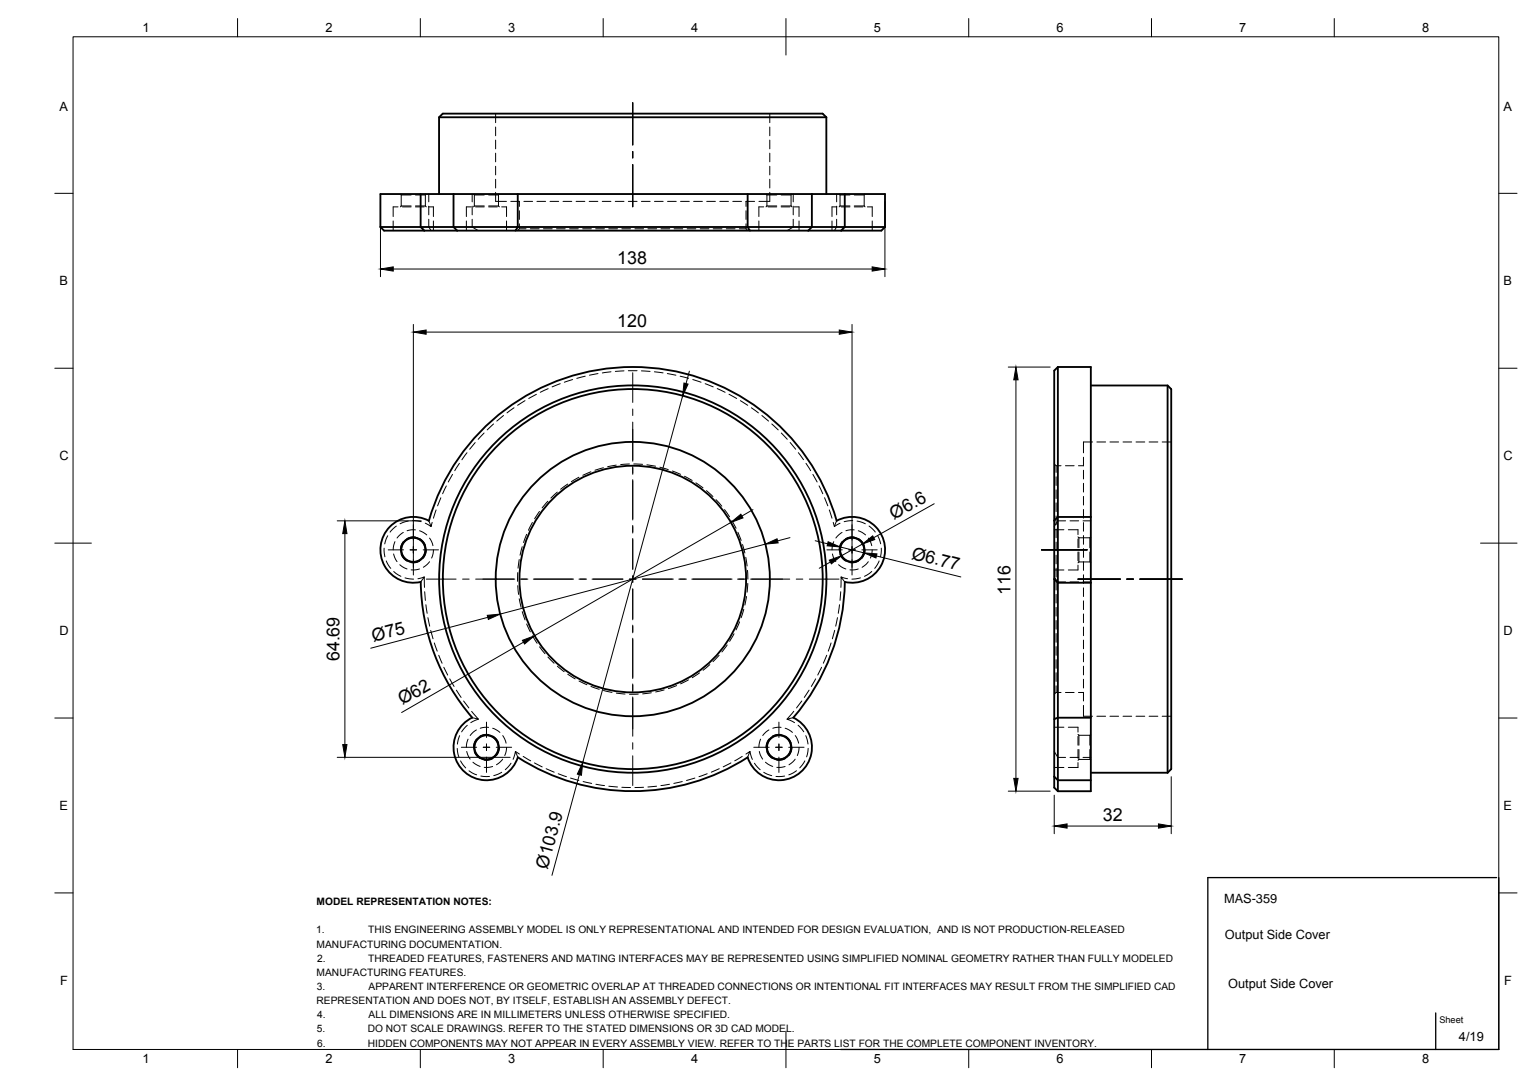
ISO-10303-21;
HEADER;
/* Generated by software containing ST-Developer
 * from STEP Tools, Inc. (www.steptools.com) 
 */

FILE_DESCRIPTION(
/* description */ (''),
/* implementation_level */ '2;1');

FILE_NAME(
/* name */ 'Output Side Cover.step',
/* time_stamp */ '2026-10-15T14:25:16-07:00',
/* author */ (''),
/* organization */ (''),
/* preprocessor_version */ 'ST-DEVELOPER v20.2',
/* originating_system */ 'Autodesk Translation Framework v15.15.0.0',
/* authorisation */ '');

FILE_SCHEMA (('AUTOMOTIVE_DESIGN { 1 0 10303 214 3 1 1 }'));
ENDSEC;

DATA;
#10=MECHANICAL_DESIGN_GEOMETRIC_PRESENTATION_REPRESENTATION('',(#324),#86429);
#288=SHAPE_REPRESENTATION_RELATIONSHIP('SRR','None',#86503,#306);
#306=ADVANCED_BREP_SHAPE_REPRESENTATION('',(#342),#86412);
#324=STYLED_ITEM('',(#86602),#342);
#342=MANIFOLD_SOLID_BREP('Body1',#15614);
#387=B_SPLINE_CURVE_WITH_KNOTS('',3,(#22589,#22590,#22591,#22592),
 .UNSPECIFIED.,.F.,.F.,(4,4),(-0.195594022319082,0.),.UNSPECIFIED.);
#388=B_SPLINE_CURVE_WITH_KNOTS('',3,(#22595,#22596,#22597,#22598),
 .UNSPECIFIED.,.F.,.F.,(4,4),(-0.195594022319045,0.),.UNSPECIFIED.);
#389=B_SPLINE_CURVE_WITH_KNOTS('',3,(#22603,#22604,#22605,#22606),
 .UNSPECIFIED.,.F.,.F.,(4,4),(-0.195594022319034,0.),.UNSPECIFIED.);
#390=B_SPLINE_CURVE_WITH_KNOTS('',3,(#22612,#22613,#22614,#22615),
 .UNSPECIFIED.,.F.,.F.,(4,4),(-0.201492965018152,0.),.UNSPECIFIED.);
#391=B_SPLINE_CURVE_WITH_KNOTS('',3,(#22621,#22622,#22623,#22624),
 .UNSPECIFIED.,.F.,.F.,(4,4),(-0.201492965018184,0.),.UNSPECIFIED.);
#392=B_SPLINE_CURVE_WITH_KNOTS('',3,(#22630,#22631,#22632,#22633),
 .UNSPECIFIED.,.F.,.F.,(4,4),(-0.201492965018239,0.),.UNSPECIFIED.);
#393=B_SPLINE_CURVE_WITH_KNOTS('',3,(#22640,#22641,#22642,#22643),
 .UNSPECIFIED.,.F.,.F.,(4,4),(-0.201492965018198,0.),.UNSPECIFIED.);
#394=B_SPLINE_CURVE_WITH_KNOTS('',3,(#22649,#22650,#22651,#22652),
 .UNSPECIFIED.,.F.,.F.,(4,4),(-0.195594022319061,0.),.UNSPECIFIED.);
#1193=CONICAL_SURFACE('',#16204,5.245,0.785398163397446);
#1194=CONICAL_SURFACE('',#16211,5.75,0.785398163397448);
#1195=CONICAL_SURFACE('',#16214,0.85,0.785398163397452);
#1196=CONICAL_SURFACE('',#16217,5.75,0.785398163397448);
#1197=CONICAL_SURFACE('',#16220,0.85,0.785398163397451);
#1198=CONICAL_SURFACE('',#16223,5.75,0.785398163397453);
#1199=CONICAL_SURFACE('',#16226,0.85,0.785398163397449);
#1200=CONICAL_SURFACE('',#16229,5.75,0.785398163397448);
#1201=CONICAL_SURFACE('',#16232,0.85,0.785398163397452);
#1202=CONICAL_SURFACE('',#16249,0.342499999999999,0.32175055439664);
#1203=CONICAL_SURFACE('',#16254,0.342499999999999,0.785398163397439);
#1204=CONICAL_SURFACE('',#16259,0.342499999999999,0.321750554396635);
#1205=CONICAL_SURFACE('',#16264,0.342499999999999,0.785398163397431);
#1206=CONICAL_SURFACE('',#16269,0.342499999999999,0.321750554396635);
#1207=CONICAL_SURFACE('',#16274,0.342499999999999,0.785398163397431);
#1208=CONICAL_SURFACE('',#16279,0.342499999999999,0.321750554396635);
#1209=CONICAL_SURFACE('',#16284,0.342499999999999,0.785398163397431);
#1210=CONICAL_SURFACE('',#16289,3.155,0.785398163397444);
#1399=CYLINDRICAL_SURFACE('',#16207,5.295);
#1400=CYLINDRICAL_SURFACE('',#16235,0.9);
#1401=CYLINDRICAL_SURFACE('',#16237,5.8);
#1402=CYLINDRICAL_SURFACE('',#16239,0.9);
#1403=CYLINDRICAL_SURFACE('',#16241,5.8);
#1404=CYLINDRICAL_SURFACE('',#16252,0.33);
#1405=CYLINDRICAL_SURFACE('',#16258,0.55);
#1406=CYLINDRICAL_SURFACE('',#16262,0.33);
#1407=CYLINDRICAL_SURFACE('',#16268,0.55);
#1408=CYLINDRICAL_SURFACE('',#16272,0.33);
#1409=CYLINDRICAL_SURFACE('',#16278,0.55);
#1410=CYLINDRICAL_SURFACE('',#16282,0.33);
#1411=CYLINDRICAL_SURFACE('',#16288,0.55);
#1412=CYLINDRICAL_SURFACE('',#16291,3.1);
#1413=CYLINDRICAL_SURFACE('',#16295,3.75);
#1414=CYLINDRICAL_SURFACE('',#16296,0.9);
#1415=CYLINDRICAL_SURFACE('',#16298,5.8);
#1416=CYLINDRICAL_SURFACE('',#16300,0.9);
#1417=CYLINDRICAL_SURFACE('',#16302,5.8);
#1652=FACE_BOUND('',#3542,.T.);
#1653=FACE_BOUND('',#3556,.T.);
#1654=FACE_BOUND('',#3557,.T.);
#1655=FACE_BOUND('',#3558,.T.);
#1656=FACE_BOUND('',#3559,.T.);
#1657=FACE_BOUND('',#3560,.T.);
#1658=FACE_BOUND('',#3565,.T.);
#1659=FACE_BOUND('',#3571,.T.);
#1660=FACE_BOUND('',#3577,.T.);
#1661=FACE_BOUND('',#3583,.T.);
#1662=FACE_BOUND('',#3588,.T.);
#1663=FACE_BOUND('',#3595,.T.);
#1664=FACE_BOUND('',#3596,.T.);
#1665=FACE_BOUND('',#3597,.T.);
#1666=FACE_BOUND('',#3598,.T.);
#1667=FACE_BOUND('',#3599,.T.);
#1889=CIRCLE('',#16205,5.295);
#1890=CIRCLE('',#16206,5.195);
#1891=CIRCLE('',#16208,5.295);
#1892=CIRCLE('',#16210,3.75);
#1893=CIRCLE('',#16212,5.7);
#1894=CIRCLE('',#16213,5.8);
#1895=CIRCLE('',#16215,0.8);
#1896=CIRCLE('',#16216,0.9);
#1897=CIRCLE('',#16218,5.7);
#1898=CIRCLE('',#16219,5.8);
#1899=CIRCLE('',#16221,0.8);
#1900=CIRCLE('',#16222,0.9);
#1901=CIRCLE('',#16224,5.7);
#1902=CIRCLE('',#16225,5.8);
#1903=CIRCLE('',#16227,0.9);
#1904=CIRCLE('',#16228,0.8);
#1905=CIRCLE('',#16230,5.8);
#1906=CIRCLE('',#16231,5.7);
#1907=CIRCLE('',#16233,0.9);
#1908=CIRCLE('',#16234,0.8);
#1909=CIRCLE('',#16236,0.9);
#1910=CIRCLE('',#16238,5.8);
#1911=CIRCLE('',#16240,0.9);
#1912=CIRCLE('',#16242,5.8);
#1913=CIRCLE('',#16244,3.15);
#1914=CIRCLE('',#16245,0.55);
#1915=CIRCLE('',#16246,0.55);
#1916=CIRCLE('',#16247,0.55);
#1917=CIRCLE('',#16248,0.55);
#1918=CIRCLE('',#16250,0.33);
#1919=CIRCLE('',#16251,0.338333333333333);
#1920=CIRCLE('',#16253,0.33);
#1921=CIRCLE('',#16255,0.355);
#1922=CIRCLE('',#16257,0.55);
#1923=CIRCLE('',#16260,0.33);
#1924=CIRCLE('',#16261,0.338333333333333);
#1925=CIRCLE('',#16263,0.33);
#1926=CIRCLE('',#16265,0.355);
#1927=CIRCLE('',#16267,0.55);
#1928=CIRCLE('',#16270,0.33);
#1929=CIRCLE('',#16271,0.338333333333333);
#1930=CIRCLE('',#16273,0.33);
#1931=CIRCLE('',#16275,0.355);
#1932=CIRCLE('',#16277,0.55);
#1933=CIRCLE('',#16280,0.33);
#1934=CIRCLE('',#16281,0.338333333333333);
#1935=CIRCLE('',#16283,0.33);
#1936=CIRCLE('',#16285,0.355);
#1937=CIRCLE('',#16287,0.55);
#1938=CIRCLE('',#16290,3.1);
#1939=CIRCLE('',#16292,3.1);
#1940=CIRCLE('',#16294,3.75);
#1941=CIRCLE('',#16297,0.9);
#1942=CIRCLE('',#16299,5.8);
#1943=CIRCLE('',#16301,0.9);
#1944=CIRCLE('',#16303,5.8);
#2617=FACE_OUTER_BOUND('',#3539,.T.);
#2618=FACE_OUTER_BOUND('',#3540,.T.);
#2619=FACE_OUTER_BOUND('',#3541,.T.);
#2620=FACE_OUTER_BOUND('',#3543,.T.);
#2621=FACE_OUTER_BOUND('',#3544,.T.);
#2622=FACE_OUTER_BOUND('',#3545,.T.);
#2623=FACE_OUTER_BOUND('',#3546,.T.);
#2624=FACE_OUTER_BOUND('',#3547,.T.);
#2625=FACE_OUTER_BOUND('',#3548,.T.);
#2626=FACE_OUTER_BOUND('',#3549,.T.);
#2627=FACE_OUTER_BOUND('',#3550,.T.);
#2628=FACE_OUTER_BOUND('',#3551,.T.);
#2629=FACE_OUTER_BOUND('',#3552,.T.);
#2630=FACE_OUTER_BOUND('',#3553,.T.);
#2631=FACE_OUTER_BOUND('',#3554,.T.);
#2632=FACE_OUTER_BOUND('',#3555,.T.);
#2633=FACE_OUTER_BOUND('',#3561,.T.);
#2634=FACE_OUTER_BOUND('',#3562,.T.);
#2635=FACE_OUTER_BOUND('',#3563,.T.);
#2636=FACE_OUTER_BOUND('',#3564,.T.);
#2637=FACE_OUTER_BOUND('',#3566,.T.);
#2638=FACE_OUTER_BOUND('',#3567,.T.);
#2639=FACE_OUTER_BOUND('',#3568,.T.);
#2640=FACE_OUTER_BOUND('',#3569,.T.);
#2641=FACE_OUTER_BOUND('',#3570,.T.);
#2642=FACE_OUTER_BOUND('',#3572,.T.);
#2643=FACE_OUTER_BOUND('',#3573,.T.);
#2644=FACE_OUTER_BOUND('',#3574,.T.);
#2645=FACE_OUTER_BOUND('',#3575,.T.);
#2646=FACE_OUTER_BOUND('',#3576,.T.);
#2647=FACE_OUTER_BOUND('',#3578,.T.);
#2648=FACE_OUTER_BOUND('',#3579,.T.);
#2649=FACE_OUTER_BOUND('',#3580,.T.);
#2650=FACE_OUTER_BOUND('',#3581,.T.);
#2651=FACE_OUTER_BOUND('',#3582,.T.);
#2652=FACE_OUTER_BOUND('',#3584,.T.);
#2653=FACE_OUTER_BOUND('',#3585,.T.);
#2654=FACE_OUTER_BOUND('',#3586,.T.);
#2655=FACE_OUTER_BOUND('',#3587,.T.);
#2656=FACE_OUTER_BOUND('',#3589,.T.);
#2657=FACE_OUTER_BOUND('',#3590,.T.);
#2658=FACE_OUTER_BOUND('',#3591,.T.);
#2659=FACE_OUTER_BOUND('',#3592,.T.);
#2660=FACE_OUTER_BOUND('',#3593,.T.);
#2661=FACE_OUTER_BOUND('',#3594,.T.);
#3539=EDGE_LOOP('',(#11021,#11022,#11023,#11024));
#3540=EDGE_LOOP('',(#11025,#11026,#11027,#11028));
#3541=EDGE_LOOP('',(#11029));
#3542=EDGE_LOOP('',(#11030));
#3543=EDGE_LOOP('',(#11031,#11032,#11033,#11034));
#3544=EDGE_LOOP('',(#11035,#11036,#11037,#11038));
#3545=EDGE_LOOP('',(#11039,#11040,#11041,#11042));
#3546=EDGE_LOOP('',(#11043,#11044,#11045,#11046));
#3547=EDGE_LOOP('',(#11047,#11048,#11049,#11050));
#3548=EDGE_LOOP('',(#11051,#11052,#11053,#11054));
#3549=EDGE_LOOP('',(#11055,#11056,#11057,#11058));
#3550=EDGE_LOOP('',(#11059,#11060,#11061,#11062));
#3551=EDGE_LOOP('',(#11063,#11064,#11065,#11066));
#3552=EDGE_LOOP('',(#11067,#11068,#11069,#11070));
#3553=EDGE_LOOP('',(#11071,#11072,#11073,#11074));
#3554=EDGE_LOOP('',(#11075,#11076,#11077,#11078));
#3555=EDGE_LOOP('',(#11079,#11080,#11081,#11082,#11083,#11084,#11085,#11086));
#3556=EDGE_LOOP('',(#11087));
#3557=EDGE_LOOP('',(#11088));
#3558=EDGE_LOOP('',(#11089));
#3559=EDGE_LOOP('',(#11090));
#3560=EDGE_LOOP('',(#11091));
#3561=EDGE_LOOP('',(#11092,#11093,#11094,#11095));
#3562=EDGE_LOOP('',(#11096,#11097,#11098,#11099));
#3563=EDGE_LOOP('',(#11100,#11101,#11102,#11103));
#3564=EDGE_LOOP('',(#11104));
#3565=EDGE_LOOP('',(#11105));
#3566=EDGE_LOOP('',(#11106,#11107,#11108,#11109));
#3567=EDGE_LOOP('',(#11110,#11111,#11112,#11113));
#3568=EDGE_LOOP('',(#11114,#11115,#11116,#11117));
#3569=EDGE_LOOP('',(#11118,#11119,#11120,#11121));
#3570=EDGE_LOOP('',(#11122));
#3571=EDGE_LOOP('',(#11123));
#3572=EDGE_LOOP('',(#11124,#11125,#11126,#11127));
#3573=EDGE_LOOP('',(#11128,#11129,#11130,#11131));
#3574=EDGE_LOOP('',(#11132,#11133,#11134,#11135));
#3575=EDGE_LOOP('',(#11136,#11137,#11138,#11139));
#3576=EDGE_LOOP('',(#11140));
#3577=EDGE_LOOP('',(#11141));
#3578=EDGE_LOOP('',(#11142,#11143,#11144,#11145));
#3579=EDGE_LOOP('',(#11146,#11147,#11148,#11149));
#3580=EDGE_LOOP('',(#11150,#11151,#11152,#11153));
#3581=EDGE_LOOP('',(#11154,#11155,#11156,#11157));
#3582=EDGE_LOOP('',(#11158));
#3583=EDGE_LOOP('',(#11159));
#3584=EDGE_LOOP('',(#11160,#11161,#11162,#11163));
#3585=EDGE_LOOP('',(#11164,#11165,#11166,#11167));
#3586=EDGE_LOOP('',(#11168,#11169,#11170,#11171));
#3587=EDGE_LOOP('',(#11172));
#3588=EDGE_LOOP('',(#11173));
#3589=EDGE_LOOP('',(#11174,#11175,#11176,#11177));
#3590=EDGE_LOOP('',(#11178,#11179,#11180,#11181));
#3591=EDGE_LOOP('',(#11182,#11183,#11184,#11185));
#3592=EDGE_LOOP('',(#11186,#11187,#11188,#11189));
#3593=EDGE_LOOP('',(#11190,#11191,#11192,#11193));
#3594=EDGE_LOOP('',(#11194,#11195,#11196,#11197,#11198,#11199,#11200,#11201));
#3595=EDGE_LOOP('',(#11202));
#3596=EDGE_LOOP('',(#11203));
#3597=EDGE_LOOP('',(#11204));
#3598=EDGE_LOOP('',(#11205));
#3599=EDGE_LOOP('',(#11206));
#4703=LINE('',#22575,#5563);
#4704=LINE('',#22579,#5564);
#4705=LINE('',#22658,#5565);
#4706=LINE('',#22661,#5566);
#4707=LINE('',#22664,#5567);
#4708=LINE('',#22668,#5568);
#4709=LINE('',#22672,#5569);
#4710=LINE('',#22689,#5570);
#4711=LINE('',#22693,#5571);
#4712=LINE('',#22697,#5572);
#4713=LINE('',#22703,#5573);
#4714=LINE('',#22708,#5574);
#4715=LINE('',#22712,#5575);
#4716=LINE('',#22716,#5576);
#4717=LINE('',#22722,#5577);
#4718=LINE('',#22727,#5578);
#4719=LINE('',#22731,#5579);
#4720=LINE('',#22735,#5580);
#4721=LINE('',#22741,#5581);
#4722=LINE('',#22746,#5582);
#4723=LINE('',#22750,#5583);
#4724=LINE('',#22754,#5584);
#4725=LINE('',#22760,#5585);
#4726=LINE('',#22764,#5586);
#4727=LINE('',#22767,#5587);
#4728=LINE('',#22773,#5588);
#4729=LINE('',#22776,#5589);
#4730=LINE('',#22780,#5590);
#4731=LINE('',#22784,#5591);
#5563=VECTOR('',#18460,5.245);
#5564=VECTOR('',#18465,5.295);
#5565=VECTOR('',#18522,1.);
#5566=VECTOR('',#18525,1.);
#5567=VECTOR('',#18528,1.);
#5568=VECTOR('',#18533,1.);
#5569=VECTOR('',#18538,1.);
#5570=VECTOR('',#18557,0.342499999999999);
#5571=VECTOR('',#18562,0.33);
#5572=VECTOR('',#18567,0.342499999999999);
#5573=VECTOR('',#18576,0.55);
#5574=VECTOR('',#18581,0.342499999999999);
#5575=VECTOR('',#18586,0.33);
#5576=VECTOR('',#18591,0.342499999999999);
#5577=VECTOR('',#18600,0.55);
#5578=VECTOR('',#18605,0.342499999999999);
#5579=VECTOR('',#18610,0.33);
#5580=VECTOR('',#18615,0.342499999999999);
#5581=VECTOR('',#18624,0.55);
#5582=VECTOR('',#18629,0.342499999999999);
#5583=VECTOR('',#18634,0.33);
#5584=VECTOR('',#18639,0.342499999999999);
#5585=VECTOR('',#18648,0.55);
#5586=VECTOR('',#18653,3.155);
#5587=VECTOR('',#18656,3.1);
#5588=VECTOR('',#18665,3.75);
#5589=VECTOR('',#18668,1.);
#5590=VECTOR('',#18673,1.);
#5591=VECTOR('',#18678,1.);
#6386=VERTEX_POINT('',#22572);
#6387=VERTEX_POINT('',#22574);
#6388=VERTEX_POINT('',#22578);
#6389=VERTEX_POINT('',#22582);
#6390=VERTEX_POINT('',#22585);
#6391=VERTEX_POINT('',#22586);
#6392=VERTEX_POINT('',#22588);
#6393=VERTEX_POINT('',#22593);
#6394=VERTEX_POINT('',#22600);
#6395=VERTEX_POINT('',#22602);
#6396=VERTEX_POINT('',#22609);
#6397=VERTEX_POINT('',#22611);
#6398=VERTEX_POINT('',#22618);
#6399=VERTEX_POINT('',#22620);
#6400=VERTEX_POINT('',#22627);
#6401=VERTEX_POINT('',#22629);
#6402=VERTEX_POINT('',#22636);
#6403=VERTEX_POINT('',#22638);
#6404=VERTEX_POINT('',#22645);
#6405=VERTEX_POINT('',#22647);
#6406=VERTEX_POINT('',#22657);
#6407=VERTEX_POINT('',#22659);
#6408=VERTEX_POINT('',#22663);
#6409=VERTEX_POINT('',#22667);
#6410=VERTEX_POINT('',#22671);
#6411=VERTEX_POINT('',#22675);
#6412=VERTEX_POINT('',#22677);
#6413=VERTEX_POINT('',#22679);
#6414=VERTEX_POINT('',#22681);
#6415=VERTEX_POINT('',#22683);
#6416=VERTEX_POINT('',#22686);
#6417=VERTEX_POINT('',#22688);
#6418=VERTEX_POINT('',#22692);
#6419=VERTEX_POINT('',#22696);
#6420=VERTEX_POINT('',#22700);
#6421=VERTEX_POINT('',#22705);
#6422=VERTEX_POINT('',#22707);
#6423=VERTEX_POINT('',#22711);
#6424=VERTEX_POINT('',#22715);
#6425=VERTEX_POINT('',#22719);
#6426=VERTEX_POINT('',#22724);
#6427=VERTEX_POINT('',#22726);
#6428=VERTEX_POINT('',#22730);
#6429=VERTEX_POINT('',#22734);
#6430=VERTEX_POINT('',#22738);
#6431=VERTEX_POINT('',#22743);
#6432=VERTEX_POINT('',#22745);
#6433=VERTEX_POINT('',#22749);
#6434=VERTEX_POINT('',#22753);
#6435=VERTEX_POINT('',#22757);
#6436=VERTEX_POINT('',#22762);
#6437=VERTEX_POINT('',#22766);
#6438=VERTEX_POINT('',#22770);
#6439=VERTEX_POINT('',#22775);
#6440=VERTEX_POINT('',#22779);
#6441=VERTEX_POINT('',#22783);
#8132=EDGE_CURVE('',#6386,#6386,#1889,.T.);
#8133=EDGE_CURVE('',#6386,#6387,#4703,.T.);
#8134=EDGE_CURVE('',#6387,#6387,#1890,.T.);
#8135=EDGE_CURVE('',#6386,#6388,#4704,.T.);
#8136=EDGE_CURVE('',#6388,#6388,#1891,.T.);
#8137=EDGE_CURVE('',#6389,#6389,#1892,.T.);
#8138=EDGE_CURVE('',#6390,#6391,#1893,.T.);
#8139=EDGE_CURVE('',#6391,#6392,#387,.T.);
#8140=EDGE_CURVE('',#6392,#6393,#1894,.T.);
#8141=EDGE_CURVE('',#6390,#6393,#388,.T.);
#8142=EDGE_CURVE('',#6391,#6394,#1895,.T.);
#8143=EDGE_CURVE('',#6394,#6395,#389,.T.);
#8144=EDGE_CURVE('',#6395,#6392,#1896,.T.);
#8145=EDGE_CURVE('',#6394,#6396,#1897,.T.);
#8146=EDGE_CURVE('',#6396,#6397,#390,.T.);
#8147=EDGE_CURVE('',#6397,#6395,#1898,.T.);
#8148=EDGE_CURVE('',#6396,#6398,#1899,.T.);
#8149=EDGE_CURVE('',#6398,#6399,#391,.T.);
#8150=EDGE_CURVE('',#6399,#6397,#1900,.T.);
#8151=EDGE_CURVE('',#6398,#6400,#1901,.T.);
#8152=EDGE_CURVE('',#6400,#6401,#392,.T.);
#8153=EDGE_CURVE('',#6401,#6399,#1902,.T.);
#8154=EDGE_CURVE('',#6402,#6401,#1903,.T.);
#8155=EDGE_CURVE('',#6400,#6403,#1904,.T.);
#8156=EDGE_CURVE('',#6403,#6402,#393,.T.);
#8157=EDGE_CURVE('',#6404,#6402,#1905,.T.);
#8158=EDGE_CURVE('',#6403,#6405,#1906,.T.);
#8159=EDGE_CURVE('',#6405,#6404,#394,.T.);
#8160=EDGE_CURVE('',#6393,#6404,#1907,.T.);
#8161=EDGE_CURVE('',#6405,#6390,#1908,.T.);
#8162=EDGE_CURVE('',#6406,#6402,#4705,.T.);
#8163=EDGE_CURVE('',#6407,#6406,#1909,.T.);
#8164=EDGE_CURVE('',#6407,#6401,#4706,.T.);
#8165=EDGE_CURVE('',#6408,#6404,#4707,.T.);
#8166=EDGE_CURVE('',#6406,#6408,#1910,.T.);
#8167=EDGE_CURVE('',#6409,#6393,#4708,.T.);
#8168=EDGE_CURVE('',#6408,#6409,#1911,.T.);
#8169=EDGE_CURVE('',#6410,#6392,#4709,.T.);
#8170=EDGE_CURVE('',#6409,#6410,#1912,.T.);
#8171=EDGE_CURVE('',#6411,#6411,#1913,.T.);
#8172=EDGE_CURVE('',#6412,#6412,#1914,.T.);
#8173=EDGE_CURVE('',#6413,#6413,#1915,.T.);
#8174=EDGE_CURVE('',#6414,#6414,#1916,.T.);
#8175=EDGE_CURVE('',#6415,#6415,#1917,.T.);
#8176=EDGE_CURVE('',#6416,#6416,#1918,.T.);
#8177=EDGE_CURVE('',#6416,#6417,#4710,.T.);
#8178=EDGE_CURVE('',#6417,#6417,#1919,.T.);
#8179=EDGE_CURVE('',#6416,#6418,#4711,.T.);
#8180=EDGE_CURVE('',#6418,#6418,#1920,.T.);
#8181=EDGE_CURVE('',#6418,#6419,#4712,.T.);
#8182=EDGE_CURVE('',#6419,#6419,#1921,.T.);
#8183=EDGE_CURVE('',#6420,#6420,#1922,.T.);
#8184=EDGE_CURVE('',#6420,#6415,#4713,.T.);
#8185=EDGE_CURVE('',#6421,#6421,#1923,.T.);
#8186=EDGE_CURVE('',#6421,#6422,#4714,.T.);
#8187=EDGE_CURVE('',#6422,#6422,#1924,.T.);
#8188=EDGE_CURVE('',#6421,#6423,#4715,.T.);
#8189=EDGE_CURVE('',#6423,#6423,#1925,.T.);
#8190=EDGE_CURVE('',#6423,#6424,#4716,.T.);
#8191=EDGE_CURVE('',#6424,#6424,#1926,.T.);
#8192=EDGE_CURVE('',#6425,#6425,#1927,.T.);
#8193=EDGE_CURVE('',#6425,#6414,#4717,.T.);
#8194=EDGE_CURVE('',#6426,#6426,#1928,.T.);
#8195=EDGE_CURVE('',#6426,#6427,#4718,.T.);
#8196=EDGE_CURVE('',#6427,#6427,#1929,.T.);
#8197=EDGE_CURVE('',#6426,#6428,#4719,.T.);
#8198=EDGE_CURVE('',#6428,#6428,#1930,.T.);
#8199=EDGE_CURVE('',#6428,#6429,#4720,.T.);
#8200=EDGE_CURVE('',#6429,#6429,#1931,.T.);
#8201=EDGE_CURVE('',#6430,#6430,#1932,.T.);
#8202=EDGE_CURVE('',#6430,#6413,#4721,.T.);
#8203=EDGE_CURVE('',#6431,#6431,#1933,.T.);
#8204=EDGE_CURVE('',#6431,#6432,#4722,.T.);
#8205=EDGE_CURVE('',#6432,#6432,#1934,.T.);
#8206=EDGE_CURVE('',#6431,#6433,#4723,.T.);
#8207=EDGE_CURVE('',#6433,#6433,#1935,.T.);
#8208=EDGE_CURVE('',#6433,#6434,#4724,.T.);
#8209=EDGE_CURVE('',#6434,#6434,#1936,.T.);
#8210=EDGE_CURVE('',#6435,#6435,#1937,.T.);
#8211=EDGE_CURVE('',#6435,#6412,#4725,.T.);
#8212=EDGE_CURVE('',#6436,#6436,#1938,.T.);
#8213=EDGE_CURVE('',#6436,#6411,#4726,.T.);
#8214=EDGE_CURVE('',#6436,#6437,#4727,.T.);
#8215=EDGE_CURVE('',#6437,#6437,#1939,.T.);
#8216=EDGE_CURVE('',#6438,#6438,#1940,.T.);
#8217=EDGE_CURVE('',#6438,#6389,#4728,.T.);
#8218=EDGE_CURVE('',#6439,#6395,#4729,.T.);
#8219=EDGE_CURVE('',#6410,#6439,#1941,.T.);
#8220=EDGE_CURVE('',#6440,#6397,#4730,.T.);
#8221=EDGE_CURVE('',#6439,#6440,#1942,.T.);
#8222=EDGE_CURVE('',#6441,#6399,#4731,.T.);
#8223=EDGE_CURVE('',#6440,#6441,#1943,.T.);
#8224=EDGE_CURVE('',#6441,#6407,#1944,.T.);
#11021=ORIENTED_EDGE('',*,*,#8132,.T.);
#11022=ORIENTED_EDGE('',*,*,#8133,.T.);
#11023=ORIENTED_EDGE('',*,*,#8134,.T.);
#11024=ORIENTED_EDGE('',*,*,#8133,.F.);
#11025=ORIENTED_EDGE('',*,*,#8132,.F.);
#11026=ORIENTED_EDGE('',*,*,#8135,.T.);
#11027=ORIENTED_EDGE('',*,*,#8136,.F.);
#11028=ORIENTED_EDGE('',*,*,#8135,.F.);
#11029=ORIENTED_EDGE('',*,*,#8134,.F.);
#11030=ORIENTED_EDGE('',*,*,#8137,.T.);
#11031=ORIENTED_EDGE('',*,*,#8138,.T.);
#11032=ORIENTED_EDGE('',*,*,#8139,.T.);
#11033=ORIENTED_EDGE('',*,*,#8140,.T.);
#11034=ORIENTED_EDGE('',*,*,#8141,.F.);
#11035=ORIENTED_EDGE('',*,*,#8142,.T.);
#11036=ORIENTED_EDGE('',*,*,#8143,.T.);
#11037=ORIENTED_EDGE('',*,*,#8144,.T.);
#11038=ORIENTED_EDGE('',*,*,#8139,.F.);
#11039=ORIENTED_EDGE('',*,*,#8145,.T.);
#11040=ORIENTED_EDGE('',*,*,#8146,.T.);
#11041=ORIENTED_EDGE('',*,*,#8147,.T.);
#11042=ORIENTED_EDGE('',*,*,#8143,.F.);
#11043=ORIENTED_EDGE('',*,*,#8148,.T.);
#11044=ORIENTED_EDGE('',*,*,#8149,.T.);
#11045=ORIENTED_EDGE('',*,*,#8150,.T.);
#11046=ORIENTED_EDGE('',*,*,#8146,.F.);
#11047=ORIENTED_EDGE('',*,*,#8151,.T.);
#11048=ORIENTED_EDGE('',*,*,#8152,.T.);
#11049=ORIENTED_EDGE('',*,*,#8153,.T.);
#11050=ORIENTED_EDGE('',*,*,#8149,.F.);
#11051=ORIENTED_EDGE('',*,*,#8154,.T.);
#11052=ORIENTED_EDGE('',*,*,#8152,.F.);
#11053=ORIENTED_EDGE('',*,*,#8155,.T.);
#11054=ORIENTED_EDGE('',*,*,#8156,.T.);
#11055=ORIENTED_EDGE('',*,*,#8157,.T.);
#11056=ORIENTED_EDGE('',*,*,#8156,.F.);
#11057=ORIENTED_EDGE('',*,*,#8158,.T.);
#11058=ORIENTED_EDGE('',*,*,#8159,.T.);
#11059=ORIENTED_EDGE('',*,*,#8160,.T.);
#11060=ORIENTED_EDGE('',*,*,#8159,.F.);
#11061=ORIENTED_EDGE('',*,*,#8161,.T.);
#11062=ORIENTED_EDGE('',*,*,#8141,.T.);
#11063=ORIENTED_EDGE('',*,*,#8154,.F.);
#11064=ORIENTED_EDGE('',*,*,#8162,.F.);
#11065=ORIENTED_EDGE('',*,*,#8163,.F.);
#11066=ORIENTED_EDGE('',*,*,#8164,.T.);
#11067=ORIENTED_EDGE('',*,*,#8157,.F.);
#11068=ORIENTED_EDGE('',*,*,#8165,.F.);
#11069=ORIENTED_EDGE('',*,*,#8166,.F.);
#11070=ORIENTED_EDGE('',*,*,#8162,.T.);
#11071=ORIENTED_EDGE('',*,*,#8160,.F.);
#11072=ORIENTED_EDGE('',*,*,#8167,.F.);
#11073=ORIENTED_EDGE('',*,*,#8168,.F.);
#11074=ORIENTED_EDGE('',*,*,#8165,.T.);
#11075=ORIENTED_EDGE('',*,*,#8140,.F.);
#11076=ORIENTED_EDGE('',*,*,#8169,.F.);
#11077=ORIENTED_EDGE('',*,*,#8170,.F.);
#11078=ORIENTED_EDGE('',*,*,#8167,.T.);
#11079=ORIENTED_EDGE('',*,*,#8138,.F.);
#11080=ORIENTED_EDGE('',*,*,#8161,.F.);
#11081=ORIENTED_EDGE('',*,*,#8158,.F.);
#11082=ORIENTED_EDGE('',*,*,#8155,.F.);
#11083=ORIENTED_EDGE('',*,*,#8151,.F.);
#11084=ORIENTED_EDGE('',*,*,#8148,.F.);
#11085=ORIENTED_EDGE('',*,*,#8145,.F.);
#11086=ORIENTED_EDGE('',*,*,#8142,.F.);
#11087=ORIENTED_EDGE('',*,*,#8171,.T.);
#11088=ORIENTED_EDGE('',*,*,#8172,.T.);
#11089=ORIENTED_EDGE('',*,*,#8173,.T.);
#11090=ORIENTED_EDGE('',*,*,#8174,.T.);
#11091=ORIENTED_EDGE('',*,*,#8175,.T.);
#11092=ORIENTED_EDGE('',*,*,#8176,.T.);
#11093=ORIENTED_EDGE('',*,*,#8177,.T.);
#11094=ORIENTED_EDGE('',*,*,#8178,.F.);
#11095=ORIENTED_EDGE('',*,*,#8177,.F.);
#11096=ORIENTED_EDGE('',*,*,#8176,.F.);
#11097=ORIENTED_EDGE('',*,*,#8179,.T.);
#11098=ORIENTED_EDGE('',*,*,#8180,.T.);
#11099=ORIENTED_EDGE('',*,*,#8179,.F.);
#11100=ORIENTED_EDGE('',*,*,#8180,.F.);
#11101=ORIENTED_EDGE('',*,*,#8181,.T.);
#11102=ORIENTED_EDGE('',*,*,#8182,.T.);
#11103=ORIENTED_EDGE('',*,*,#8181,.F.);
#11104=ORIENTED_EDGE('',*,*,#8183,.T.);
#11105=ORIENTED_EDGE('',*,*,#8182,.F.);
#11106=ORIENTED_EDGE('',*,*,#8183,.F.);
#11107=ORIENTED_EDGE('',*,*,#8184,.T.);
#11108=ORIENTED_EDGE('',*,*,#8175,.F.);
#11109=ORIENTED_EDGE('',*,*,#8184,.F.);
#11110=ORIENTED_EDGE('',*,*,#8185,.T.);
#11111=ORIENTED_EDGE('',*,*,#8186,.T.);
#11112=ORIENTED_EDGE('',*,*,#8187,.F.);
#11113=ORIENTED_EDGE('',*,*,#8186,.F.);
#11114=ORIENTED_EDGE('',*,*,#8185,.F.);
#11115=ORIENTED_EDGE('',*,*,#8188,.T.);
#11116=ORIENTED_EDGE('',*,*,#8189,.T.);
#11117=ORIENTED_EDGE('',*,*,#8188,.F.);
#11118=ORIENTED_EDGE('',*,*,#8189,.F.);
#11119=ORIENTED_EDGE('',*,*,#8190,.T.);
#11120=ORIENTED_EDGE('',*,*,#8191,.T.);
#11121=ORIENTED_EDGE('',*,*,#8190,.F.);
#11122=ORIENTED_EDGE('',*,*,#8192,.T.);
#11123=ORIENTED_EDGE('',*,*,#8191,.F.);
#11124=ORIENTED_EDGE('',*,*,#8192,.F.);
#11125=ORIENTED_EDGE('',*,*,#8193,.T.);
#11126=ORIENTED_EDGE('',*,*,#8174,.F.);
#11127=ORIENTED_EDGE('',*,*,#8193,.F.);
#11128=ORIENTED_EDGE('',*,*,#8194,.T.);
#11129=ORIENTED_EDGE('',*,*,#8195,.T.);
#11130=ORIENTED_EDGE('',*,*,#8196,.F.);
#11131=ORIENTED_EDGE('',*,*,#8195,.F.);
#11132=ORIENTED_EDGE('',*,*,#8194,.F.);
#11133=ORIENTED_EDGE('',*,*,#8197,.T.);
#11134=ORIENTED_EDGE('',*,*,#8198,.T.);
#11135=ORIENTED_EDGE('',*,*,#8197,.F.);
#11136=ORIENTED_EDGE('',*,*,#8198,.F.);
#11137=ORIENTED_EDGE('',*,*,#8199,.T.);
#11138=ORIENTED_EDGE('',*,*,#8200,.T.);
#11139=ORIENTED_EDGE('',*,*,#8199,.F.);
#11140=ORIENTED_EDGE('',*,*,#8201,.T.);
#11141=ORIENTED_EDGE('',*,*,#8200,.F.);
#11142=ORIENTED_EDGE('',*,*,#8201,.F.);
#11143=ORIENTED_EDGE('',*,*,#8202,.T.);
#11144=ORIENTED_EDGE('',*,*,#8173,.F.);
#11145=ORIENTED_EDGE('',*,*,#8202,.F.);
#11146=ORIENTED_EDGE('',*,*,#8203,.T.);
#11147=ORIENTED_EDGE('',*,*,#8204,.T.);
#11148=ORIENTED_EDGE('',*,*,#8205,.F.);
#11149=ORIENTED_EDGE('',*,*,#8204,.F.);
#11150=ORIENTED_EDGE('',*,*,#8203,.F.);
#11151=ORIENTED_EDGE('',*,*,#8206,.T.);
#11152=ORIENTED_EDGE('',*,*,#8207,.T.);
#11153=ORIENTED_EDGE('',*,*,#8206,.F.);
#11154=ORIENTED_EDGE('',*,*,#8207,.F.);
#11155=ORIENTED_EDGE('',*,*,#8208,.T.);
#11156=ORIENTED_EDGE('',*,*,#8209,.T.);
#11157=ORIENTED_EDGE('',*,*,#8208,.F.);
#11158=ORIENTED_EDGE('',*,*,#8210,.T.);
#11159=ORIENTED_EDGE('',*,*,#8209,.F.);
#11160=ORIENTED_EDGE('',*,*,#8210,.F.);
#11161=ORIENTED_EDGE('',*,*,#8211,.T.);
#11162=ORIENTED_EDGE('',*,*,#8172,.F.);
#11163=ORIENTED_EDGE('',*,*,#8211,.F.);
#11164=ORIENTED_EDGE('',*,*,#8212,.T.);
#11165=ORIENTED_EDGE('',*,*,#8213,.T.);
#11166=ORIENTED_EDGE('',*,*,#8171,.F.);
#11167=ORIENTED_EDGE('',*,*,#8213,.F.);
#11168=ORIENTED_EDGE('',*,*,#8212,.F.);
#11169=ORIENTED_EDGE('',*,*,#8214,.T.);
#11170=ORIENTED_EDGE('',*,*,#8215,.T.);
#11171=ORIENTED_EDGE('',*,*,#8214,.F.);
#11172=ORIENTED_EDGE('',*,*,#8216,.T.);
#11173=ORIENTED_EDGE('',*,*,#8215,.F.);
#11174=ORIENTED_EDGE('',*,*,#8216,.F.);
#11175=ORIENTED_EDGE('',*,*,#8217,.T.);
#11176=ORIENTED_EDGE('',*,*,#8137,.F.);
#11177=ORIENTED_EDGE('',*,*,#8217,.F.);
#11178=ORIENTED_EDGE('',*,*,#8144,.F.);
#11179=ORIENTED_EDGE('',*,*,#8218,.F.);
#11180=ORIENTED_EDGE('',*,*,#8219,.F.);
#11181=ORIENTED_EDGE('',*,*,#8169,.T.);
#11182=ORIENTED_EDGE('',*,*,#8147,.F.);
#11183=ORIENTED_EDGE('',*,*,#8220,.F.);
#11184=ORIENTED_EDGE('',*,*,#8221,.F.);
#11185=ORIENTED_EDGE('',*,*,#8218,.T.);
#11186=ORIENTED_EDGE('',*,*,#8150,.F.);
#11187=ORIENTED_EDGE('',*,*,#8222,.F.);
#11188=ORIENTED_EDGE('',*,*,#8223,.F.);
#11189=ORIENTED_EDGE('',*,*,#8220,.T.);
#11190=ORIENTED_EDGE('',*,*,#8153,.F.);
#11191=ORIENTED_EDGE('',*,*,#8164,.F.);
#11192=ORIENTED_EDGE('',*,*,#8224,.F.);
#11193=ORIENTED_EDGE('',*,*,#8222,.T.);
#11194=ORIENTED_EDGE('',*,*,#8224,.T.);
#11195=ORIENTED_EDGE('',*,*,#8163,.T.);
#11196=ORIENTED_EDGE('',*,*,#8166,.T.);
#11197=ORIENTED_EDGE('',*,*,#8168,.T.);
#11198=ORIENTED_EDGE('',*,*,#8170,.T.);
#11199=ORIENTED_EDGE('',*,*,#8219,.T.);
#11200=ORIENTED_EDGE('',*,*,#8221,.T.);
#11201=ORIENTED_EDGE('',*,*,#8223,.T.);
#11202=ORIENTED_EDGE('',*,*,#8178,.T.);
#11203=ORIENTED_EDGE('',*,*,#8187,.T.);
#11204=ORIENTED_EDGE('',*,*,#8196,.T.);
#11205=ORIENTED_EDGE('',*,*,#8205,.T.);
#11206=ORIENTED_EDGE('',*,*,#8136,.T.);
#14595=PLANE('',#16209);
#14596=PLANE('',#16243);
#14597=PLANE('',#16256);
#14598=PLANE('',#16266);
#14599=PLANE('',#16276);
#14600=PLANE('',#16286);
#14601=PLANE('',#16293);
#14602=PLANE('',#16304);
#14973=ADVANCED_FACE('',(#2617),#1193,.T.);
#14974=ADVANCED_FACE('',(#2618),#1399,.T.);
#14975=ADVANCED_FACE('',(#2619,#1652),#14595,.T.);
#14976=ADVANCED_FACE('',(#2620),#1194,.T.);
#14977=ADVANCED_FACE('',(#2621),#1195,.T.);
#14978=ADVANCED_FACE('',(#2622),#1196,.T.);
#14979=ADVANCED_FACE('',(#2623),#1197,.T.);
#14980=ADVANCED_FACE('',(#2624),#1198,.T.);
#14981=ADVANCED_FACE('',(#2625),#1199,.T.);
#14982=ADVANCED_FACE('',(#2626),#1200,.T.);
#14983=ADVANCED_FACE('',(#2627),#1201,.T.);
#14984=ADVANCED_FACE('',(#2628),#1400,.T.);
#14985=ADVANCED_FACE('',(#2629),#1401,.T.);
#14986=ADVANCED_FACE('',(#2630),#1402,.T.);
#14987=ADVANCED_FACE('',(#2631),#1403,.T.);
#14988=ADVANCED_FACE('',(#2632,#1653,#1654,#1655,#1656,#1657),#14596,.F.);
#14989=ADVANCED_FACE('',(#2633),#1202,.F.);
#14990=ADVANCED_FACE('',(#2634),#1404,.F.);
#14991=ADVANCED_FACE('',(#2635),#1203,.F.);
#14992=ADVANCED_FACE('',(#2636,#1658),#14597,.F.);
#14993=ADVANCED_FACE('',(#2637),#1405,.F.);
#14994=ADVANCED_FACE('',(#2638),#1204,.F.);
#14995=ADVANCED_FACE('',(#2639),#1406,.F.);
#14996=ADVANCED_FACE('',(#2640),#1205,.F.);
#14997=ADVANCED_FACE('',(#2641,#1659),#14598,.F.);
#14998=ADVANCED_FACE('',(#2642),#1407,.F.);
#14999=ADVANCED_FACE('',(#2643),#1206,.F.);
#15000=ADVANCED_FACE('',(#2644),#1408,.F.);
#15001=ADVANCED_FACE('',(#2645),#1207,.F.);
#15002=ADVANCED_FACE('',(#2646,#1660),#14599,.F.);
#15003=ADVANCED_FACE('',(#2647),#1409,.F.);
#15004=ADVANCED_FACE('',(#2648),#1208,.F.);
#15005=ADVANCED_FACE('',(#2649),#1410,.F.);
#15006=ADVANCED_FACE('',(#2650),#1209,.F.);
#15007=ADVANCED_FACE('',(#2651,#1661),#14600,.F.);
#15008=ADVANCED_FACE('',(#2652),#1411,.F.);
#15009=ADVANCED_FACE('',(#2653),#1210,.F.);
#15010=ADVANCED_FACE('',(#2654),#1412,.F.);
#15011=ADVANCED_FACE('',(#2655,#1662),#14601,.F.);
#15012=ADVANCED_FACE('',(#2656),#1413,.F.);
#15013=ADVANCED_FACE('',(#2657),#1414,.T.);
#15014=ADVANCED_FACE('',(#2658),#1415,.T.);
#15015=ADVANCED_FACE('',(#2659),#1416,.T.);
#15016=ADVANCED_FACE('',(#2660),#1417,.T.);
#15017=ADVANCED_FACE('',(#2661,#1663,#1664,#1665,#1666,#1667),#14602,.T.);
#15614=CLOSED_SHELL('',(#14973,#14974,#14975,#14976,#14977,#14978,#14979,
#14980,#14981,#14982,#14983,#14984,#14985,#14986,#14987,#14988,#14989,#14990,
#14991,#14992,#14993,#14994,#14995,#14996,#14997,#14998,#14999,#15000,#15001,
#15002,#15003,#15004,#15005,#15006,#15007,#15008,#15009,#15010,#15011,#15012,
#15013,#15014,#15015,#15016,#15017));
#16203=AXIS2_PLACEMENT_3D('',#22570,#18454,#18455);
#16204=AXIS2_PLACEMENT_3D('',#22571,#18456,#18457);
#16205=AXIS2_PLACEMENT_3D('',#22573,#18458,#18459);
#16206=AXIS2_PLACEMENT_3D('',#22576,#18461,#18462);
#16207=AXIS2_PLACEMENT_3D('',#22577,#18463,#18464);
#16208=AXIS2_PLACEMENT_3D('',#22580,#18466,#18467);
#16209=AXIS2_PLACEMENT_3D('',#22581,#18468,#18469);
#16210=AXIS2_PLACEMENT_3D('',#22583,#18470,#18471);
#16211=AXIS2_PLACEMENT_3D('',#22584,#18472,#18473);
#16212=AXIS2_PLACEMENT_3D('',#22587,#18474,#18475);
#16213=AXIS2_PLACEMENT_3D('',#22594,#18476,#18477);
#16214=AXIS2_PLACEMENT_3D('',#22599,#18478,#18479);
#16215=AXIS2_PLACEMENT_3D('',#22601,#18480,#18481);
#16216=AXIS2_PLACEMENT_3D('',#22607,#18482,#18483);
#16217=AXIS2_PLACEMENT_3D('',#22608,#18484,#18485);
#16218=AXIS2_PLACEMENT_3D('',#22610,#18486,#18487);
#16219=AXIS2_PLACEMENT_3D('',#22616,#18488,#18489);
#16220=AXIS2_PLACEMENT_3D('',#22617,#18490,#18491);
#16221=AXIS2_PLACEMENT_3D('',#22619,#18492,#18493);
#16222=AXIS2_PLACEMENT_3D('',#22625,#18494,#18495);
#16223=AXIS2_PLACEMENT_3D('',#22626,#18496,#18497);
#16224=AXIS2_PLACEMENT_3D('',#22628,#18498,#18499);
#16225=AXIS2_PLACEMENT_3D('',#22634,#18500,#18501);
#16226=AXIS2_PLACEMENT_3D('',#22635,#18502,#18503);
#16227=AXIS2_PLACEMENT_3D('',#22637,#18504,#18505);
#16228=AXIS2_PLACEMENT_3D('',#22639,#18506,#18507);
#16229=AXIS2_PLACEMENT_3D('',#22644,#18508,#18509);
#16230=AXIS2_PLACEMENT_3D('',#22646,#18510,#18511);
#16231=AXIS2_PLACEMENT_3D('',#22648,#18512,#18513);
#16232=AXIS2_PLACEMENT_3D('',#22653,#18514,#18515);
#16233=AXIS2_PLACEMENT_3D('',#22654,#18516,#18517);
#16234=AXIS2_PLACEMENT_3D('',#22655,#18518,#18519);
#16235=AXIS2_PLACEMENT_3D('',#22656,#18520,#18521);
#16236=AXIS2_PLACEMENT_3D('',#22660,#18523,#18524);
#16237=AXIS2_PLACEMENT_3D('',#22662,#18526,#18527);
#16238=AXIS2_PLACEMENT_3D('',#22665,#18529,#18530);
#16239=AXIS2_PLACEMENT_3D('',#22666,#18531,#18532);
#16240=AXIS2_PLACEMENT_3D('',#22669,#18534,#18535);
#16241=AXIS2_PLACEMENT_3D('',#22670,#18536,#18537);
#16242=AXIS2_PLACEMENT_3D('',#22673,#18539,#18540);
#16243=AXIS2_PLACEMENT_3D('',#22674,#18541,#18542);
#16244=AXIS2_PLACEMENT_3D('',#22676,#18543,#18544);
#16245=AXIS2_PLACEMENT_3D('',#22678,#18545,#18546);
#16246=AXIS2_PLACEMENT_3D('',#22680,#18547,#18548);
#16247=AXIS2_PLACEMENT_3D('',#22682,#18549,#18550);
#16248=AXIS2_PLACEMENT_3D('',#22684,#18551,#18552);
#16249=AXIS2_PLACEMENT_3D('',#22685,#18553,#18554);
#16250=AXIS2_PLACEMENT_3D('',#22687,#18555,#18556);
#16251=AXIS2_PLACEMENT_3D('',#22690,#18558,#18559);
#16252=AXIS2_PLACEMENT_3D('',#22691,#18560,#18561);
#16253=AXIS2_PLACEMENT_3D('',#22694,#18563,#18564);
#16254=AXIS2_PLACEMENT_3D('',#22695,#18565,#18566);
#16255=AXIS2_PLACEMENT_3D('',#22698,#18568,#18569);
#16256=AXIS2_PLACEMENT_3D('',#22699,#18570,#18571);
#16257=AXIS2_PLACEMENT_3D('',#22701,#18572,#18573);
#16258=AXIS2_PLACEMENT_3D('',#22702,#18574,#18575);
#16259=AXIS2_PLACEMENT_3D('',#22704,#18577,#18578);
#16260=AXIS2_PLACEMENT_3D('',#22706,#18579,#18580);
#16261=AXIS2_PLACEMENT_3D('',#22709,#18582,#18583);
#16262=AXIS2_PLACEMENT_3D('',#22710,#18584,#18585);
#16263=AXIS2_PLACEMENT_3D('',#22713,#18587,#18588);
#16264=AXIS2_PLACEMENT_3D('',#22714,#18589,#18590);
#16265=AXIS2_PLACEMENT_3D('',#22717,#18592,#18593);
#16266=AXIS2_PLACEMENT_3D('',#22718,#18594,#18595);
#16267=AXIS2_PLACEMENT_3D('',#22720,#18596,#18597);
#16268=AXIS2_PLACEMENT_3D('',#22721,#18598,#18599);
#16269=AXIS2_PLACEMENT_3D('',#22723,#18601,#18602);
#16270=AXIS2_PLACEMENT_3D('',#22725,#18603,#18604);
#16271=AXIS2_PLACEMENT_3D('',#22728,#18606,#18607);
#16272=AXIS2_PLACEMENT_3D('',#22729,#18608,#18609);
#16273=AXIS2_PLACEMENT_3D('',#22732,#18611,#18612);
#16274=AXIS2_PLACEMENT_3D('',#22733,#18613,#18614);
#16275=AXIS2_PLACEMENT_3D('',#22736,#18616,#18617);
#16276=AXIS2_PLACEMENT_3D('',#22737,#18618,#18619);
#16277=AXIS2_PLACEMENT_3D('',#22739,#18620,#18621);
#16278=AXIS2_PLACEMENT_3D('',#22740,#18622,#18623);
#16279=AXIS2_PLACEMENT_3D('',#22742,#18625,#18626);
#16280=AXIS2_PLACEMENT_3D('',#22744,#18627,#18628);
#16281=AXIS2_PLACEMENT_3D('',#22747,#18630,#18631);
#16282=AXIS2_PLACEMENT_3D('',#22748,#18632,#18633);
#16283=AXIS2_PLACEMENT_3D('',#22751,#18635,#18636);
#16284=AXIS2_PLACEMENT_3D('',#22752,#18637,#18638);
#16285=AXIS2_PLACEMENT_3D('',#22755,#18640,#18641);
#16286=AXIS2_PLACEMENT_3D('',#22756,#18642,#18643);
#16287=AXIS2_PLACEMENT_3D('',#22758,#18644,#18645);
#16288=AXIS2_PLACEMENT_3D('',#22759,#18646,#18647);
#16289=AXIS2_PLACEMENT_3D('',#22761,#18649,#18650);
#16290=AXIS2_PLACEMENT_3D('',#22763,#18651,#18652);
#16291=AXIS2_PLACEMENT_3D('',#22765,#18654,#18655);
#16292=AXIS2_PLACEMENT_3D('',#22768,#18657,#18658);
#16293=AXIS2_PLACEMENT_3D('',#22769,#18659,#18660);
#16294=AXIS2_PLACEMENT_3D('',#22771,#18661,#18662);
#16295=AXIS2_PLACEMENT_3D('',#22772,#18663,#18664);
#16296=AXIS2_PLACEMENT_3D('',#22774,#18666,#18667);
#16297=AXIS2_PLACEMENT_3D('',#22777,#18669,#18670);
#16298=AXIS2_PLACEMENT_3D('',#22778,#18671,#18672);
#16299=AXIS2_PLACEMENT_3D('',#22781,#18674,#18675);
#16300=AXIS2_PLACEMENT_3D('',#22782,#18676,#18677);
#16301=AXIS2_PLACEMENT_3D('',#22785,#18679,#18680);
#16302=AXIS2_PLACEMENT_3D('',#22786,#18681,#18682);
#16303=AXIS2_PLACEMENT_3D('',#22787,#18683,#18684);
#16304=AXIS2_PLACEMENT_3D('',#22788,#18685,#18686);
#18454=DIRECTION('axis',(0.,0.,1.));
#18455=DIRECTION('refdir',(1.,0.,0.));
#18456=DIRECTION('center_axis',(0.,-1.,0.));
#18457=DIRECTION('ref_axis',(1.,0.,0.));
#18458=DIRECTION('center_axis',(0.,1.,0.));
#18459=DIRECTION('ref_axis',(1.,0.,0.));
#18460=DIRECTION('',(0.707106781186546,0.707106781186549,8.65956056235491E-17));
#18461=DIRECTION('center_axis',(0.,-1.,0.));
#18462=DIRECTION('ref_axis',(1.,0.,0.));
#18463=DIRECTION('center_axis',(0.,1.,0.));
#18464=DIRECTION('ref_axis',(1.,0.,0.));
#18465=DIRECTION('',(0.,-1.,0.));
#18466=DIRECTION('center_axis',(0.,-1.,0.));
#18467=DIRECTION('ref_axis',(1.,0.,0.));
#18468=DIRECTION('center_axis',(0.,1.,0.));
#18469=DIRECTION('ref_axis',(1.,0.,0.));
#18470=DIRECTION('center_axis',(0.,-1.,0.));
#18471=DIRECTION('ref_axis',(0.,0.,1.));
#18472=DIRECTION('center_axis',(0.,1.,0.));
#18473=DIRECTION('ref_axis',(1.,0.,0.));
#18474=DIRECTION('center_axis',(0.,1.,0.));
#18475=DIRECTION('ref_axis',(1.,0.,0.));
#18476=DIRECTION('center_axis',(0.,-1.,0.));
#18477=DIRECTION('ref_axis',(1.,0.,0.));
#18478=DIRECTION('center_axis',(0.,1.,0.));
#18479=DIRECTION('ref_axis',(1.,0.,0.));
#18480=DIRECTION('center_axis',(0.,1.,0.));
#18481=DIRECTION('ref_axis',(1.,0.,0.));
#18482=DIRECTION('center_axis',(0.,-1.,0.));
#18483=DIRECTION('ref_axis',(1.,0.,0.));
#18484=DIRECTION('center_axis',(0.,1.,0.));
#18485=DIRECTION('ref_axis',(1.,0.,0.));
#18486=DIRECTION('center_axis',(0.,1.,0.));
#18487=DIRECTION('ref_axis',(1.,0.,0.));
#18488=DIRECTION('center_axis',(0.,-1.,0.));
#18489=DIRECTION('ref_axis',(1.,0.,0.));
#18490=DIRECTION('center_axis',(0.,1.,0.));
#18491=DIRECTION('ref_axis',(1.,0.,0.));
#18492=DIRECTION('center_axis',(0.,1.,0.));
#18493=DIRECTION('ref_axis',(1.,0.,0.));
#18494=DIRECTION('center_axis',(0.,-1.,0.));
#18495=DIRECTION('ref_axis',(1.,0.,0.));
#18496=DIRECTION('center_axis',(0.,1.,0.));
#18497=DIRECTION('ref_axis',(1.,0.,0.));
#18498=DIRECTION('center_axis',(0.,1.,0.));
#18499=DIRECTION('ref_axis',(1.,0.,0.));
#18500=DIRECTION('center_axis',(0.,-1.,0.));
#18501=DIRECTION('ref_axis',(1.,0.,0.));
#18502=DIRECTION('center_axis',(0.,1.,0.));
#18503=DIRECTION('ref_axis',(-1.,0.,0.));
#18504=DIRECTION('center_axis',(0.,-1.,0.));
#18505=DIRECTION('ref_axis',(-1.,0.,0.));
#18506=DIRECTION('center_axis',(0.,1.,0.));
#18507=DIRECTION('ref_axis',(-1.,0.,0.));
#18508=DIRECTION('center_axis',(0.,1.,0.));
#18509=DIRECTION('ref_axis',(-1.,0.,0.));
#18510=DIRECTION('center_axis',(0.,-1.,0.));
#18511=DIRECTION('ref_axis',(-1.,0.,0.));
#18512=DIRECTION('center_axis',(0.,1.,0.));
#18513=DIRECTION('ref_axis',(-1.,0.,0.));
#18514=DIRECTION('center_axis',(0.,1.,0.));
#18515=DIRECTION('ref_axis',(-1.,0.,0.));
#18516=DIRECTION('center_axis',(0.,-1.,0.));
#18517=DIRECTION('ref_axis',(-1.,0.,0.));
#18518=DIRECTION('center_axis',(0.,1.,0.));
#18519=DIRECTION('ref_axis',(-1.,0.,0.));
#18520=DIRECTION('center_axis',(0.,-1.,0.));
#18521=DIRECTION('ref_axis',(-0.656178714924787,0.,-0.754605522163505));
#18522=DIRECTION('',(0.,-1.,0.));
#18523=DIRECTION('center_axis',(0.,1.,0.));
#18524=DIRECTION('ref_axis',(1.,0.,0.));
#18525=DIRECTION('',(0.,-1.,0.));
#18526=DIRECTION('center_axis',(0.,-1.,0.));
#18527=DIRECTION('ref_axis',(1.,0.,0.));
#18528=DIRECTION('',(0.,-1.,0.));
#18529=DIRECTION('center_axis',(0.,1.,0.));
#18530=DIRECTION('ref_axis',(1.,0.,0.));
#18531=DIRECTION('center_axis',(0.,-1.,0.));
#18532=DIRECTION('ref_axis',(-0.991227900682635,0.,0.132163720091017));
#18533=DIRECTION('',(0.,-1.,0.));
#18534=DIRECTION('center_axis',(0.,1.,0.));
#18535=DIRECTION('ref_axis',(1.,0.,0.));
#18536=DIRECTION('center_axis',(0.,-1.,0.));
#18537=DIRECTION('ref_axis',(1.,0.,0.));
#18538=DIRECTION('',(0.,-1.,0.));
#18539=DIRECTION('center_axis',(0.,1.,0.));
#18540=DIRECTION('ref_axis',(1.,0.,0.));
#18541=DIRECTION('center_axis',(0.,1.,0.));
#18542=DIRECTION('ref_axis',(1.,0.,0.));
#18543=DIRECTION('center_axis',(0.,1.,0.));
#18544=DIRECTION('ref_axis',(0.,0.,1.));
#18545=DIRECTION('center_axis',(0.,1.,0.));
#18546=DIRECTION('ref_axis',(1.,0.,0.));
#18547=DIRECTION('center_axis',(0.,1.,0.));
#18548=DIRECTION('ref_axis',(1.,0.,0.));
#18549=DIRECTION('center_axis',(0.,1.,0.));
#18550=DIRECTION('ref_axis',(1.,0.,0.));
#18551=DIRECTION('center_axis',(0.,1.,0.));
#18552=DIRECTION('ref_axis',(1.,0.,0.));
#18553=DIRECTION('center_axis',(0.,1.,0.));
#18554=DIRECTION('ref_axis',(1.,0.,0.));
#18555=DIRECTION('center_axis',(0.,-1.,0.));
#18556=DIRECTION('ref_axis',(1.,0.,0.));
#18557=DIRECTION('',(-0.316227766016836,0.948683298050514,3.87267321454036E-17));
#18558=DIRECTION('center_axis',(0.,-1.,0.));
#18559=DIRECTION('ref_axis',(1.,0.,0.));
#18560=DIRECTION('center_axis',(0.,-1.,0.));
#18561=DIRECTION('ref_axis',(1.,0.,0.));
#18562=DIRECTION('',(0.,-1.,0.));
#18563=DIRECTION('center_axis',(0.,-1.,0.));
#18564=DIRECTION('ref_axis',(1.,0.,0.));
#18565=DIRECTION('center_axis',(0.,-1.,0.));
#18566=DIRECTION('ref_axis',(1.,0.,0.));
#18567=DIRECTION('',(-0.707106781186541,-0.707106781186554,-8.65956056235485E-17));
#18568=DIRECTION('center_axis',(0.,-1.,0.));
#18569=DIRECTION('ref_axis',(1.,0.,0.));
#18570=DIRECTION('center_axis',(0.,1.,0.));
#18571=DIRECTION('ref_axis',(0.,0.,1.));
#18572=DIRECTION('center_axis',(0.,-1.,0.));
#18573=DIRECTION('ref_axis',(1.,0.,0.));
#18574=DIRECTION('center_axis',(0.,-1.,0.));
#18575=DIRECTION('ref_axis',(1.,0.,0.));
#18576=DIRECTION('',(0.,-1.,0.));
#18577=DIRECTION('center_axis',(0.,1.,0.));
#18578=DIRECTION('ref_axis',(1.,0.,0.));
#18579=DIRECTION('center_axis',(0.,-1.,0.));
#18580=DIRECTION('ref_axis',(1.,0.,0.));
#18581=DIRECTION('',(-0.316227766016831,0.948683298050516,3.8726732145403E-17));
#18582=DIRECTION('center_axis',(0.,-1.,0.));
#18583=DIRECTION('ref_axis',(1.,0.,0.));
#18584=DIRECTION('center_axis',(0.,-1.,0.));
#18585=DIRECTION('ref_axis',(1.,0.,0.));
#18586=DIRECTION('',(0.,-1.,0.));
#18587=DIRECTION('center_axis',(0.,-1.,0.));
#18588=DIRECTION('ref_axis',(1.,0.,0.));
#18589=DIRECTION('center_axis',(0.,-1.,0.));
#18590=DIRECTION('ref_axis',(1.,0.,0.));
#18591=DIRECTION('',(-0.707106781186535,-0.70710678118656,-8.65956056235478E-17));
#18592=DIRECTION('center_axis',(0.,-1.,0.));
#18593=DIRECTION('ref_axis',(1.,0.,0.));
#18594=DIRECTION('center_axis',(0.,1.,0.));
#18595=DIRECTION('ref_axis',(0.,0.,1.));
#18596=DIRECTION('center_axis',(0.,-1.,0.));
#18597=DIRECTION('ref_axis',(1.,0.,0.));
#18598=DIRECTION('center_axis',(0.,-1.,0.));
#18599=DIRECTION('ref_axis',(1.,0.,0.));
#18600=DIRECTION('',(0.,-1.,0.));
#18601=DIRECTION('center_axis',(0.,1.,0.));
#18602=DIRECTION('ref_axis',(1.,0.,0.));
#18603=DIRECTION('center_axis',(0.,-1.,0.));
#18604=DIRECTION('ref_axis',(1.,0.,0.));
#18605=DIRECTION('',(-0.316227766016831,0.948683298050516,3.8726732145403E-17));
#18606=DIRECTION('center_axis',(0.,-1.,0.));
#18607=DIRECTION('ref_axis',(1.,0.,0.));
#18608=DIRECTION('center_axis',(0.,-1.,0.));
#18609=DIRECTION('ref_axis',(1.,0.,0.));
#18610=DIRECTION('',(0.,-1.,0.));
#18611=DIRECTION('center_axis',(0.,-1.,0.));
#18612=DIRECTION('ref_axis',(1.,0.,0.));
#18613=DIRECTION('center_axis',(0.,-1.,0.));
#18614=DIRECTION('ref_axis',(1.,0.,0.));
#18615=DIRECTION('',(-0.707106781186535,-0.70710678118656,-8.65956056235478E-17));
#18616=DIRECTION('center_axis',(0.,-1.,0.));
#18617=DIRECTION('ref_axis',(1.,0.,0.));
#18618=DIRECTION('center_axis',(0.,1.,0.));
#18619=DIRECTION('ref_axis',(0.,0.,1.));
#18620=DIRECTION('center_axis',(0.,-1.,0.));
#18621=DIRECTION('ref_axis',(1.,0.,0.));
#18622=DIRECTION('center_axis',(0.,-1.,0.));
#18623=DIRECTION('ref_axis',(1.,0.,0.));
#18624=DIRECTION('',(0.,-1.,0.));
#18625=DIRECTION('center_axis',(0.,1.,0.));
#18626=DIRECTION('ref_axis',(1.,0.,0.));
#18627=DIRECTION('center_axis',(0.,-1.,0.));
#18628=DIRECTION('ref_axis',(1.,0.,0.));
#18629=DIRECTION('',(-0.316227766016831,0.948683298050516,3.8726732145403E-17));
#18630=DIRECTION('center_axis',(0.,-1.,0.));
#18631=DIRECTION('ref_axis',(1.,0.,0.));
#18632=DIRECTION('center_axis',(0.,-1.,0.));
#18633=DIRECTION('ref_axis',(1.,0.,0.));
#18634=DIRECTION('',(0.,-1.,0.));
#18635=DIRECTION('center_axis',(0.,-1.,0.));
#18636=DIRECTION('ref_axis',(1.,0.,0.));
#18637=DIRECTION('center_axis',(0.,-1.,0.));
#18638=DIRECTION('ref_axis',(1.,0.,0.));
#18639=DIRECTION('',(-0.707106781186535,-0.70710678118656,-8.65956056235478E-17));
#18640=DIRECTION('center_axis',(0.,-1.,0.));
#18641=DIRECTION('ref_axis',(1.,0.,0.));
#18642=DIRECTION('center_axis',(0.,1.,0.));
#18643=DIRECTION('ref_axis',(0.,0.,1.));
#18644=DIRECTION('center_axis',(0.,-1.,0.));
#18645=DIRECTION('ref_axis',(1.,0.,0.));
#18646=DIRECTION('center_axis',(0.,-1.,0.));
#18647=DIRECTION('ref_axis',(1.,0.,0.));
#18648=DIRECTION('',(0.,-1.,0.));
#18649=DIRECTION('center_axis',(0.,-1.,0.));
#18650=DIRECTION('ref_axis',(0.,0.,1.));
#18651=DIRECTION('center_axis',(0.,1.,0.));
#18652=DIRECTION('ref_axis',(1.,0.,0.));
#18653=DIRECTION('',(8.65956056235489E-17,-0.70710678118655,-0.707106781186544));
#18654=DIRECTION('center_axis',(0.,1.,0.));
#18655=DIRECTION('ref_axis',(0.,0.,1.));
#18656=DIRECTION('',(0.,1.,0.));
#18657=DIRECTION('center_axis',(0.,1.,0.));
#18658=DIRECTION('ref_axis',(1.,0.,0.));
#18659=DIRECTION('center_axis',(0.,-1.,0.));
#18660=DIRECTION('ref_axis',(0.,0.,-1.));
#18661=DIRECTION('center_axis',(0.,1.,0.));
#18662=DIRECTION('ref_axis',(1.,0.,0.));
#18663=DIRECTION('center_axis',(0.,1.,0.));
#18664=DIRECTION('ref_axis',(0.,0.,1.));
#18665=DIRECTION('',(0.,1.,0.));
#18666=DIRECTION('center_axis',(0.,-1.,0.));
#18667=DIRECTION('ref_axis',(1.,0.,0.));
#18668=DIRECTION('',(0.,-1.,0.));
#18669=DIRECTION('center_axis',(0.,1.,0.));
#18670=DIRECTION('ref_axis',(1.,0.,0.));
#18671=DIRECTION('center_axis',(0.,-1.,0.));
#18672=DIRECTION('ref_axis',(1.,0.,0.));
#18673=DIRECTION('',(0.,-1.,0.));
#18674=DIRECTION('center_axis',(0.,1.,0.));
#18675=DIRECTION('ref_axis',(1.,0.,0.));
#18676=DIRECTION('center_axis',(0.,-1.,0.));
#18677=DIRECTION('ref_axis',(1.,0.,0.));
#18678=DIRECTION('',(0.,-1.,0.));
#18679=DIRECTION('center_axis',(0.,1.,0.));
#18680=DIRECTION('ref_axis',(1.,0.,0.));
#18681=DIRECTION('center_axis',(0.,-1.,0.));
#18682=DIRECTION('ref_axis',(1.,0.,0.));
#18683=DIRECTION('center_axis',(0.,1.,0.));
#18684=DIRECTION('ref_axis',(1.,0.,0.));
#18685=DIRECTION('center_axis',(0.,1.,0.));
#18686=DIRECTION('ref_axis',(1.,0.,0.));
#22570=CARTESIAN_POINT('',(0.,0.,0.));
#22571=CARTESIAN_POINT('Origin',(0.,-2.45,7.2));
#22572=CARTESIAN_POINT('',(-5.295,-2.5,7.2));
#22573=CARTESIAN_POINT('Origin',(0.,-2.5,7.2));
#22574=CARTESIAN_POINT('',(-5.195,-2.4,7.2));
#22575=CARTESIAN_POINT('',(-5.245,-2.45,7.2));
#22576=CARTESIAN_POINT('Origin',(0.,-2.4,7.2));
#22577=CARTESIAN_POINT('Origin',(0.,-4.6,7.2));
#22578=CARTESIAN_POINT('',(-5.295,-4.6,7.2));
#22579=CARTESIAN_POINT('',(-5.295,-4.6,7.2));
#22580=CARTESIAN_POINT('Origin',(0.,-4.6,7.2));
#22581=CARTESIAN_POINT('Origin',(0.,-2.4,7.2));
#22582=CARTESIAN_POINT('',(4.59242549680257E-16,-2.4,3.45));
#22583=CARTESIAN_POINT('Origin',(0.,-2.4,7.2));
#22584=CARTESIAN_POINT('Origin',(0.,-5.55,7.2));
#22585=CARTESIAN_POINT('',(-5.51591157610535,-5.6,8.63691317920985));
#22586=CARTESIAN_POINT('',(5.51591157610535,-5.6,8.63691317920985));
#22587=CARTESIAN_POINT('Origin',(0.,-5.6,7.2));
#22588=CARTESIAN_POINT('',(5.57660788571496,-5.5,8.79419085713778));
#22589=CARTESIAN_POINT('Ctrl Pts',(5.51591157610535,-5.6,8.63691317920985));
#22590=CARTESIAN_POINT('Ctrl Pts',(5.53455522536305,-5.56837145414589,8.69081065313349));
#22591=CARTESIAN_POINT('Ctrl Pts',(5.55504723137092,-5.53469693041622,8.74337706591871));
#22592=CARTESIAN_POINT('Ctrl Pts',(5.57660788571496,-5.5,8.79419085713778));
#22593=CARTESIAN_POINT('',(-5.57660788571496,-5.5,8.79419085713778));
#22594=CARTESIAN_POINT('Origin',(0.,-5.5,7.2));
#22595=CARTESIAN_POINT('Ctrl Pts',(-5.51591157610535,-5.6,8.63691317920985));
#22596=CARTESIAN_POINT('Ctrl Pts',(-5.53455522536305,-5.56837145414589,
8.6908106531335));
#22597=CARTESIAN_POINT('Ctrl Pts',(-5.55504723137093,-5.53469693041621,
8.74337706591873));
#22598=CARTESIAN_POINT('Ctrl Pts',(-5.57660788571496,-5.5,8.79419085713778));
#22599=CARTESIAN_POINT('Origin',(6.,-5.55,8.));
#22600=CARTESIAN_POINT('',(5.69969977760644,-5.6,7.25850166795172));
#22601=CARTESIAN_POINT('Origin',(6.,-5.6,8.));
#22602=CARTESIAN_POINT('',(5.79948381734181,-5.5,7.12262136993645));
#22603=CARTESIAN_POINT('Ctrl Pts',(5.69969977760644,-5.6,7.25850166795172));
#22604=CARTESIAN_POINT('Ctrl Pts',(5.73181372922814,-5.56837145414589,7.21137187414533));
#22605=CARTESIAN_POINT('Ctrl Pts',(5.76536271654192,-5.53469693041621,7.16601092713632));
#22606=CARTESIAN_POINT('Ctrl Pts',(5.79948381734181,-5.5,7.12262136993645));
#22607=CARTESIAN_POINT('Origin',(6.,-5.5,8.));
#22608=CARTESIAN_POINT('Origin',(0.,-5.55,7.2));
#22609=CARTESIAN_POINT('',(4.22058574132406,-5.6,3.36898760115136));
#22610=CARTESIAN_POINT('Origin',(0.,-5.6,7.2));
#22611=CARTESIAN_POINT('',(4.39098268679659,-5.5,3.41063711895356));
#22612=CARTESIAN_POINT('Ctrl Pts',(4.22058574132406,-5.6,3.36898760115136));
#22613=CARTESIAN_POINT('Ctrl Pts',(4.27772143963444,-5.56861968092285,3.38524395544776));
#22614=CARTESIAN_POINT('Ctrl Pts',(4.33480274427804,-5.53491157572283,3.39897341264218));
#22615=CARTESIAN_POINT('Ctrl Pts',(4.39098268679659,-5.5,3.41063711895356));
#22616=CARTESIAN_POINT('Origin',(0.,-5.5,7.2));
#22617=CARTESIAN_POINT('Origin',(4.,-5.55,2.6));
#22618=CARTESIAN_POINT('',(3.20783191206668,-5.6,2.48833209744929));
#22619=CARTESIAN_POINT('Origin',(4.,-5.6,2.6));
#22620=CARTESIAN_POINT('',(3.14292474054464,-5.5,2.32536933960403));
#22621=CARTESIAN_POINT('Ctrl Pts',(3.20783191206668,-5.6,2.48833209744929));
#22622=CARTESIAN_POINT('Ctrl Pts',(3.18379924141574,-5.56861968092285,2.43400726134454));
#22623=CARTESIAN_POINT('Ctrl Pts',(3.16227654075062,-5.53491157572284,2.37938540957487));
#22624=CARTESIAN_POINT('Ctrl Pts',(3.14292474054464,-5.5,2.32536933960403));
#22625=CARTESIAN_POINT('Origin',(4.,-5.5,2.6));
#22626=CARTESIAN_POINT('Origin',(0.,-5.55,7.2));
#22627=CARTESIAN_POINT('',(-3.20783191206668,-5.6,2.48833209744929));
#22628=CARTESIAN_POINT('Origin',(0.,-5.6,7.2));
#22629=CARTESIAN_POINT('',(-3.14292474054464,-5.5,2.32536933960403));
#22630=CARTESIAN_POINT('Ctrl Pts',(-3.20783191206668,-5.6,2.48833209744929));
#22631=CARTESIAN_POINT('Ctrl Pts',(-3.18379924141574,-5.56861968092285,
2.43400726134455));
#22632=CARTESIAN_POINT('Ctrl Pts',(-3.16227654075063,-5.53491157572285,
2.37938540957488));
#22633=CARTESIAN_POINT('Ctrl Pts',(-3.14292474054464,-5.5,2.32536933960403));
#22634=CARTESIAN_POINT('Origin',(0.,-5.5,7.2));
#22635=CARTESIAN_POINT('Origin',(-4.,-5.55,2.6));
#22636=CARTESIAN_POINT('',(-4.39098268679659,-5.5,3.41063711895356));
#22637=CARTESIAN_POINT('Origin',(-4.,-5.5,2.6));
#22638=CARTESIAN_POINT('',(-4.22058574132406,-5.6,3.36898760115135));
#22639=CARTESIAN_POINT('Origin',(-4.,-5.6,2.6));
#22640=CARTESIAN_POINT('Ctrl Pts',(-4.22058574132406,-5.6,3.36898760115136));
#22641=CARTESIAN_POINT('Ctrl Pts',(-4.27772143963443,-5.56861968092285,
3.38524395544776));
#22642=CARTESIAN_POINT('Ctrl Pts',(-4.33480274427803,-5.53491157572284,
3.39897341264218));
#22643=CARTESIAN_POINT('Ctrl Pts',(-4.39098268679659,-5.5,3.41063711895356));
#22644=CARTESIAN_POINT('Origin',(0.,-5.55,7.2));
#22645=CARTESIAN_POINT('',(-5.79948381734181,-5.5,7.12262136993645));
#22646=CARTESIAN_POINT('Origin',(0.,-5.5,7.2));
#22647=CARTESIAN_POINT('',(-5.69969977760644,-5.6,7.25850166795172));
#22648=CARTESIAN_POINT('Origin',(0.,-5.6,7.2));
#22649=CARTESIAN_POINT('Ctrl Pts',(-5.69969977760644,-5.6,7.25850166795172));
#22650=CARTESIAN_POINT('Ctrl Pts',(-5.73181372922814,-5.56837145414589,
7.21137187414533));
#22651=CARTESIAN_POINT('Ctrl Pts',(-5.76536271654191,-5.53469693041622,
7.16601092713633));
#22652=CARTESIAN_POINT('Ctrl Pts',(-5.79948381734181,-5.5,7.12262136993645));
#22653=CARTESIAN_POINT('Origin',(-6.,-5.55,8.));
#22654=CARTESIAN_POINT('Origin',(-6.,-5.5,8.));
#22655=CARTESIAN_POINT('Origin',(-6.,-5.6,8.));
#22656=CARTESIAN_POINT('Origin',(-4.,-4.6,2.6));
#22657=CARTESIAN_POINT('',(-4.39098268679659,-4.6,3.41063711895356));
#22658=CARTESIAN_POINT('',(-4.39098268679659,-4.6,3.41063711895356));
#22659=CARTESIAN_POINT('',(-3.14292474054464,-4.6,2.32536933960403));
#22660=CARTESIAN_POINT('Origin',(-4.,-4.6,2.6));
#22661=CARTESIAN_POINT('',(-3.14292474054464,-4.6,2.32536933960403));
#22662=CARTESIAN_POINT('Origin',(0.,-4.6,7.2));
#22663=CARTESIAN_POINT('',(-5.79948381734181,-4.6,7.12262136993645));
#22664=CARTESIAN_POINT('',(-5.79948381734181,-4.6,7.12262136993645));
#22665=CARTESIAN_POINT('Origin',(0.,-4.6,7.2));
#22666=CARTESIAN_POINT('Origin',(-6.,-4.6,8.));
#22667=CARTESIAN_POINT('',(-5.57660788571496,-4.6,8.79419085713778));
#22668=CARTESIAN_POINT('',(-5.57660788571496,-4.6,8.79419085713778));
#22669=CARTESIAN_POINT('Origin',(-6.,-4.6,8.));
#22670=CARTESIAN_POINT('Origin',(0.,-4.6,7.2));
#22671=CARTESIAN_POINT('',(5.57660788571496,-4.6,8.79419085713778));
#22672=CARTESIAN_POINT('',(5.57660788571496,-4.6,8.79419085713778));
#22673=CARTESIAN_POINT('Origin',(0.,-4.6,7.2));
#22674=CARTESIAN_POINT('Origin',(0.,-5.6,7.2));
#22675=CARTESIAN_POINT('',(-3.85763741731416E-16,-5.6,4.05));
#22676=CARTESIAN_POINT('Origin',(0.,-5.6,7.2));
#22677=CARTESIAN_POINT('',(5.45,-5.6,8.));
#22678=CARTESIAN_POINT('Origin',(6.,-5.6,8.));
#22679=CARTESIAN_POINT('',(-6.55,-5.6,8.));
#22680=CARTESIAN_POINT('Origin',(-6.,-5.6,8.));
#22681=CARTESIAN_POINT('',(3.45,-5.6,2.6));
#22682=CARTESIAN_POINT('Origin',(4.,-5.6,2.6));
#22683=CARTESIAN_POINT('',(-4.55,-5.6,2.6));
#22684=CARTESIAN_POINT('Origin',(-4.,-5.6,2.6));
#22685=CARTESIAN_POINT('Origin',(-4.,-4.5875,2.6));
#22686=CARTESIAN_POINT('',(-4.33,-4.625,2.6));
#22687=CARTESIAN_POINT('Origin',(-4.,-4.625,2.6));
#22688=CARTESIAN_POINT('',(-4.33833333333333,-4.6,2.6));
#22689=CARTESIAN_POINT('',(-4.3425,-4.5875,2.6));
#22690=CARTESIAN_POINT('Origin',(-4.,-4.6,2.6));
#22691=CARTESIAN_POINT('Origin',(-4.,-4.775,2.6));
#22692=CARTESIAN_POINT('',(-4.33,-4.925,2.6));
#22693=CARTESIAN_POINT('',(-4.33,-4.775,2.6));
#22694=CARTESIAN_POINT('Origin',(-4.,-4.925,2.6));
#22695=CARTESIAN_POINT('Origin',(-4.,-4.9375,2.6));
#22696=CARTESIAN_POINT('',(-4.355,-4.95,2.6));
#22697=CARTESIAN_POINT('',(-4.3425,-4.9375,2.6));
#22698=CARTESIAN_POINT('Origin',(-4.,-4.95,2.6));
#22699=CARTESIAN_POINT('Origin',(-3.45,-4.95,2.6));
#22700=CARTESIAN_POINT('',(-4.55,-4.95,2.6));
#22701=CARTESIAN_POINT('Origin',(-4.,-4.95,2.6));
#22702=CARTESIAN_POINT('Origin',(-4.,-5.275,2.6));
#22703=CARTESIAN_POINT('',(-4.55,-5.275,2.6));
#22704=CARTESIAN_POINT('Origin',(4.,-4.5875,2.6));
#22705=CARTESIAN_POINT('',(3.67,-4.625,2.6));
#22706=CARTESIAN_POINT('Origin',(4.,-4.625,2.6));
#22707=CARTESIAN_POINT('',(3.66166666666667,-4.6,2.6));
#22708=CARTESIAN_POINT('',(3.6575,-4.5875,2.6));
#22709=CARTESIAN_POINT('Origin',(4.,-4.6,2.6));
#22710=CARTESIAN_POINT('Origin',(4.,-4.775,2.6));
#22711=CARTESIAN_POINT('',(3.67,-4.925,2.6));
#22712=CARTESIAN_POINT('',(3.67,-4.775,2.6));
#22713=CARTESIAN_POINT('Origin',(4.,-4.925,2.6));
#22714=CARTESIAN_POINT('Origin',(4.,-4.9375,2.6));
#22715=CARTESIAN_POINT('',(3.645,-4.95,2.6));
#22716=CARTESIAN_POINT('',(3.6575,-4.9375,2.6));
#22717=CARTESIAN_POINT('Origin',(4.,-4.95,2.6));
#22718=CARTESIAN_POINT('Origin',(4.55,-4.95,2.6));
#22719=CARTESIAN_POINT('',(3.45,-4.95,2.6));
#22720=CARTESIAN_POINT('Origin',(4.,-4.95,2.6));
#22721=CARTESIAN_POINT('Origin',(4.,-5.275,2.6));
#22722=CARTESIAN_POINT('',(3.45,-5.275,2.6));
#22723=CARTESIAN_POINT('Origin',(-6.,-4.5875,8.));
#22724=CARTESIAN_POINT('',(-6.33,-4.625,8.));
#22725=CARTESIAN_POINT('Origin',(-6.,-4.625,8.));
#22726=CARTESIAN_POINT('',(-6.33833333333333,-4.6,8.));
#22727=CARTESIAN_POINT('',(-6.3425,-4.5875,8.));
#22728=CARTESIAN_POINT('Origin',(-6.,-4.6,8.));
#22729=CARTESIAN_POINT('Origin',(-6.,-4.775,8.));
#22730=CARTESIAN_POINT('',(-6.33,-4.925,8.));
#22731=CARTESIAN_POINT('',(-6.33,-4.775,8.));
#22732=CARTESIAN_POINT('Origin',(-6.,-4.925,8.));
#22733=CARTESIAN_POINT('Origin',(-6.,-4.9375,8.));
#22734=CARTESIAN_POINT('',(-6.355,-4.95,8.));
#22735=CARTESIAN_POINT('',(-6.3425,-4.9375,8.));
#22736=CARTESIAN_POINT('Origin',(-6.,-4.95,8.));
#22737=CARTESIAN_POINT('Origin',(-5.45,-4.95,8.));
#22738=CARTESIAN_POINT('',(-6.55,-4.95,8.));
#22739=CARTESIAN_POINT('Origin',(-6.,-4.95,8.));
#22740=CARTESIAN_POINT('Origin',(-6.,-5.275,8.));
#22741=CARTESIAN_POINT('',(-6.55,-5.275,8.));
#22742=CARTESIAN_POINT('Origin',(6.,-4.5875,8.));
#22743=CARTESIAN_POINT('',(5.67,-4.625,8.));
#22744=CARTESIAN_POINT('Origin',(6.,-4.625,8.));
#22745=CARTESIAN_POINT('',(5.66166666666667,-4.6,8.));
#22746=CARTESIAN_POINT('',(5.6575,-4.5875,8.));
#22747=CARTESIAN_POINT('Origin',(6.,-4.6,8.));
#22748=CARTESIAN_POINT('Origin',(6.,-4.775,8.));
#22749=CARTESIAN_POINT('',(5.67,-4.925,8.));
#22750=CARTESIAN_POINT('',(5.67,-4.775,8.));
#22751=CARTESIAN_POINT('Origin',(6.,-4.925,8.));
#22752=CARTESIAN_POINT('Origin',(6.,-4.9375,8.));
#22753=CARTESIAN_POINT('',(5.645,-4.95,8.));
#22754=CARTESIAN_POINT('',(5.6575,-4.9375,8.));
#22755=CARTESIAN_POINT('Origin',(6.,-4.95,8.));
#22756=CARTESIAN_POINT('Origin',(6.55,-4.95,8.));
#22757=CARTESIAN_POINT('',(5.45,-4.95,8.));
#22758=CARTESIAN_POINT('Origin',(6.,-4.95,8.));
#22759=CARTESIAN_POINT('Origin',(6.,-5.275,8.));
#22760=CARTESIAN_POINT('',(5.45,-5.275,8.));
#22761=CARTESIAN_POINT('Origin',(0.,-5.605,7.2));
#22762=CARTESIAN_POINT('',(-3.79640507735679E-16,-5.55,4.1));
#22763=CARTESIAN_POINT('Origin',(0.,-5.55,7.2));
#22764=CARTESIAN_POINT('',(3.8637606513099E-16,-5.605,4.045));
#22765=CARTESIAN_POINT('Origin',(0.,-5.175,7.2));
#22766=CARTESIAN_POINT('',(-3.7964050773568E-16,-4.8,4.1));
#22767=CARTESIAN_POINT('',(-3.79640507735679E-16,-5.175,4.1));
#22768=CARTESIAN_POINT('Origin',(0.,-4.8,7.2));
#22769=CARTESIAN_POINT('Origin',(0.,-4.8,10.95));
#22770=CARTESIAN_POINT('',(-4.59242549680257E-16,-4.8,3.45));
#22771=CARTESIAN_POINT('Origin',(0.,-4.8,7.2));
#22772=CARTESIAN_POINT('Origin',(0.,-3.55,7.2));
#22773=CARTESIAN_POINT('',(-4.59242549680257E-16,-3.55,3.45));
#22774=CARTESIAN_POINT('Origin',(6.,-4.6,8.));
#22775=CARTESIAN_POINT('',(5.79948381734181,-4.6,7.12262136993645));
#22776=CARTESIAN_POINT('',(5.79948381734181,-4.6,7.12262136993645));
#22777=CARTESIAN_POINT('Origin',(6.,-4.6,8.));
#22778=CARTESIAN_POINT('Origin',(0.,-4.6,7.2));
#22779=CARTESIAN_POINT('',(4.39098268679659,-4.6,3.41063711895356));
#22780=CARTESIAN_POINT('',(4.39098268679659,-4.6,3.41063711895356));
#22781=CARTESIAN_POINT('Origin',(0.,-4.6,7.2));
#22782=CARTESIAN_POINT('Origin',(4.,-4.6,2.6));
#22783=CARTESIAN_POINT('',(3.14292474054464,-4.6,2.32536933960403));
#22784=CARTESIAN_POINT('',(3.14292474054464,-4.6,2.32536933960403));
#22785=CARTESIAN_POINT('Origin',(4.,-4.6,2.6));
#22786=CARTESIAN_POINT('Origin',(0.,-4.6,7.2));
#22787=CARTESIAN_POINT('Origin',(0.,-4.6,7.2));
#22788=CARTESIAN_POINT('Origin',(0.,-4.6,7.2));
#86392=UNCERTAINTY_MEASURE_WITH_UNIT(LENGTH_MEASURE(0.001),#86430,
'DISTANCE_ACCURACY_VALUE',
'Maximum model space distance between geometric entities at asserted c
onnectivities');
#86409=UNCERTAINTY_MEASURE_WITH_UNIT(LENGTH_MEASURE(0.001),#86430,
'DISTANCE_ACCURACY_VALUE',
'Maximum model space distance between geometric entities at asserted c
onnectivities');
#86412=(
GEOMETRIC_REPRESENTATION_CONTEXT(3)
GLOBAL_UNCERTAINTY_ASSIGNED_CONTEXT((#86392))
GLOBAL_UNIT_ASSIGNED_CONTEXT((#86430,#86432,#86433))
REPRESENTATION_CONTEXT('','3D')
);
#86429=(
GEOMETRIC_REPRESENTATION_CONTEXT(3)
GLOBAL_UNCERTAINTY_ASSIGNED_CONTEXT((#86409))
GLOBAL_UNIT_ASSIGNED_CONTEXT((#86430,#86432,#86433))
REPRESENTATION_CONTEXT('','3D')
);
#86430=(
LENGTH_UNIT()
NAMED_UNIT(*)
SI_UNIT(.CENTI.,.METRE.)
);
#86432=(
NAMED_UNIT(*)
PLANE_ANGLE_UNIT()
SI_UNIT($,.RADIAN.)
);
#86433=(
NAMED_UNIT(*)
SI_UNIT($,.STERADIAN.)
SOLID_ANGLE_UNIT()
);
#86436=SHAPE_DEFINITION_REPRESENTATION(#86455,#86503);
#86455=PRODUCT_DEFINITION_SHAPE('',$,#86523);
#86503=SHAPE_REPRESENTATION('',(#16203),#86412);
#86520=PRODUCT_DEFINITION_CONTEXT('part definition',#86579,'design');
#86523=PRODUCT_DEFINITION('Output Side Cover','Output Side Cover',#86542,
#86520);
#86542=PRODUCT_DEFINITION_FORMATION('',$,#86583);
#86579=APPLICATION_CONTEXT(
'Core Data for Automotive Mechanical Design Process');
#86580=PRODUCT_CONTEXT('part definition',#86579,'mechanical');
#86583=PRODUCT('Output Side Cover','Output Side Cover',$,(#86580));
#86602=PRESENTATION_STYLE_ASSIGNMENT((#86620));
#86620=SURFACE_STYLE_USAGE(.BOTH.,#86638);
#86638=SURFACE_SIDE_STYLE('',(#86656));
#86656=SURFACE_STYLE_FILL_AREA(#86674);
#86674=FILL_AREA_STYLE('Opaque(184,188,192)',(#86692));
#86692=FILL_AREA_STYLE_COLOUR('Opaque(184,188,192)',#86710);
#86710=COLOUR_RGB('Opaque(184,188,192)', 0.66274510, 0.83137255, 0.94901961);
ENDSEC;
END-ISO-10303-21;
